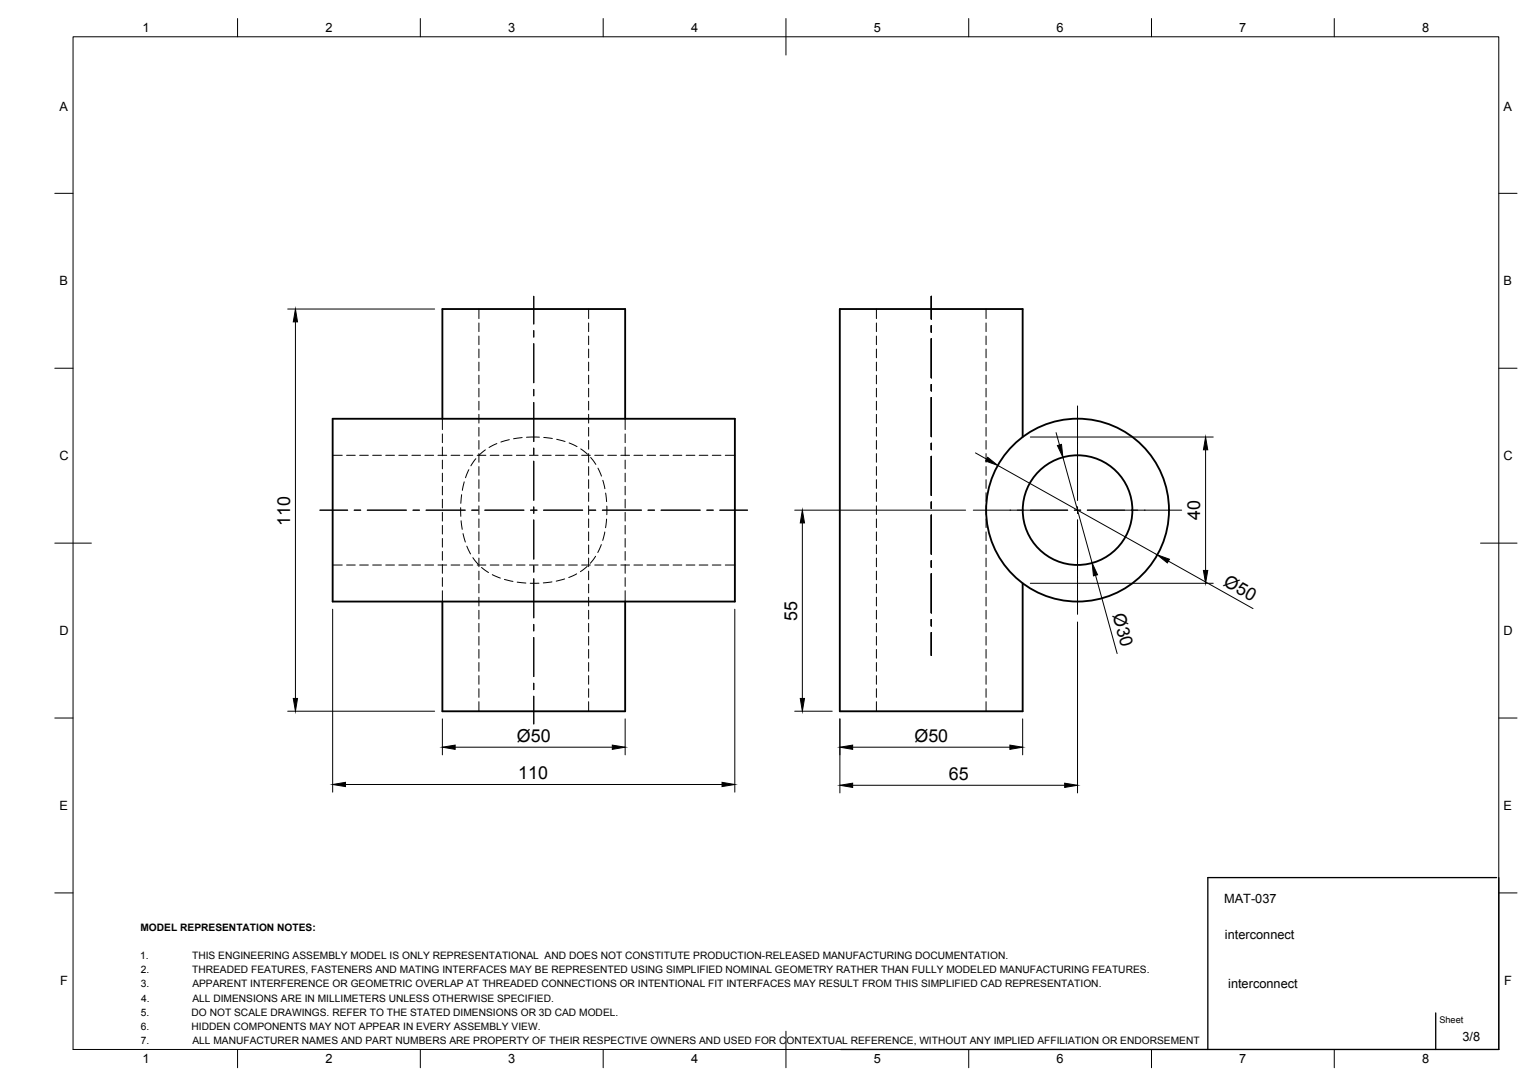
ISO-10303-21;
HEADER;
/* Generated by software containing ST-Developer
 * from STEP Tools, Inc. (www.steptools.com) 
 */

FILE_DESCRIPTION(
/* description */ ('STEP AP214'),
/* implementation_level */ '2;1');

FILE_NAME(
/* name */ 'interconnect.step',
/* time_stamp */ '2026-11-14T21:09:07-08:00',
/* author */ (''),
/* organization */ (''),
/* preprocessor_version */ 'ST-DEVELOPER v20.2',
/* originating_system */ 'Autodesk Translation Framework v15.17.0.0',
/* authorisation */ '');

FILE_SCHEMA (('AUTOMOTIVE_DESIGN { 1 0 10303 214 3 1 1 }'));
ENDSEC;

DATA;
#10=MECHANICAL_DESIGN_GEOMETRIC_PRESENTATION_REPRESENTATION('',(#78),#2059);
#64=SHAPE_REPRESENTATION_RELATIONSHIP('SRR','None',#2094,#71);
#71=ADVANCED_BREP_SHAPE_REPRESENTATION('',(#85),#2052);
#78=STYLED_ITEM('',(#2138),#85);
#85=MANIFOLD_SOLID_BREP('Body1',#975);
#92=PLANE('',#1074);
#93=PLANE('',#1075);
#94=PLANE('',#1076);
#95=PLANE('',#1077);
#125=FACE_BOUND('',#214,.T.);
#126=FACE_BOUND('',#217,.T.);
#127=FACE_BOUND('',#219,.T.);
#128=FACE_BOUND('',#221,.T.);
#129=FACE_BOUND('',#223,.T.);
#130=FACE_BOUND('',#225,.T.);
#145=B_SPLINE_CURVE_WITH_KNOTS('',3,(#1500,#1501,#1502,#1503,#1504,#1505,
#1506,#1507,#1508,#1509,#1510,#1511,#1512,#1513,#1514,#1515,#1516,#1517,
#1518,#1519,#1520,#1521,#1522,#1523,#1524,#1525,#1526,#1527,#1528,#1529,
#1530,#1531,#1532,#1533,#1534,#1535,#1536,#1537,#1538,#1539,#1540,#1541,
#1542,#1543,#1544,#1545,#1546,#1547,#1548,#1549,#1550,#1551,#1552,#1553,
#1554,#1555,#1556,#1557,#1558,#1559,#1560,#1561,#1562,#1563,#1564,#1565),
 .UNSPECIFIED.,.T.,.F.,(4,2,2,2,2,2,2,2,2,2,2,2,2,2,2,2,2,2,2,2,2,2,2,2,
2,2,2,2,2,2,2,2,4),(-13.1042885251054,-12.7312036729648,-12.3581188208242,
-11.9850339686836,-11.611949116543,-11.2858660599115,-10.95978300328,-10.3939996985545,
-9.82821639382906,-9.2624330891036,-8.69664978437814,-8.37056672774664,
-8.04448367111514,-7.67139881897453,-7.29831396683392,-6.92522911469332,
-6.55214426255271,-6.1790594104121,-5.80597455827149,-5.43288970613088,
-5.05980485399027,-4.73372179735877,-4.40763874072727,-3.84185543600181,
-3.27607213127635,-2.7102888265509,-2.14450552182544,-1.81842246519393,
-1.49233940856243,-1.11925455642182,-0.746169704281216,-0.373084852140608,
0.),.UNSPECIFIED.);
#156=FACE_OUTER_BOUND('',#212,.T.);
#157=FACE_OUTER_BOUND('',#213,.T.);
#158=FACE_OUTER_BOUND('',#215,.T.);
#159=FACE_OUTER_BOUND('',#216,.T.);
#160=FACE_OUTER_BOUND('',#218,.T.);
#161=FACE_OUTER_BOUND('',#220,.T.);
#162=FACE_OUTER_BOUND('',#222,.T.);
#163=FACE_OUTER_BOUND('',#224,.T.);
#212=EDGE_LOOP('',(#659,#660,#661,#662));
#213=EDGE_LOOP('',(#663,#664,#665,#666));
#214=EDGE_LOOP('',(#667));
#215=EDGE_LOOP('',(#668,#669,#670,#671));
#216=EDGE_LOOP('',(#672,#673,#674,#675));
#217=EDGE_LOOP('',(#676));
#218=EDGE_LOOP('',(#677));
#219=EDGE_LOOP('',(#678));
#220=EDGE_LOOP('',(#679));
#221=EDGE_LOOP('',(#680));
#222=EDGE_LOOP('',(#681));
#223=EDGE_LOOP('',(#682));
#224=EDGE_LOOP('',(#683));
#225=EDGE_LOOP('',(#684));
#288=LINE('',#1491,#353);
#289=LINE('',#1497,#354);
#290=LINE('',#1570,#355);
#291=LINE('',#1576,#356);
#353=VECTOR('',#1188,15.);
#354=VECTOR('',#1195,25.);
#355=VECTOR('',#1202,15.);
#356=VECTOR('',#1209,25.);
#418=CIRCLE('',#1063,15.);
#419=CIRCLE('',#1064,15.);
#420=CIRCLE('',#1066,25.);
#421=CIRCLE('',#1067,25.);
#422=CIRCLE('',#1069,15.);
#423=CIRCLE('',#1070,15.);
#424=CIRCLE('',#1072,25.);
#425=CIRCLE('',#1073,25.);
#461=VERTEX_POINT('',#1488);
#462=VERTEX_POINT('',#1490);
#463=VERTEX_POINT('',#1494);
#464=VERTEX_POINT('',#1496);
#465=VERTEX_POINT('',#1499);
#466=VERTEX_POINT('',#1567);
#467=VERTEX_POINT('',#1569);
#468=VERTEX_POINT('',#1573);
#469=VERTEX_POINT('',#1575);
#540=EDGE_CURVE('',#461,#461,#418,.T.);
#541=EDGE_CURVE('',#461,#462,#288,.T.);
#542=EDGE_CURVE('',#462,#462,#419,.T.);
#543=EDGE_CURVE('',#463,#463,#420,.T.);
#544=EDGE_CURVE('',#463,#464,#289,.T.);
#545=EDGE_CURVE('',#464,#464,#421,.T.);
#546=EDGE_CURVE('',#465,#465,#145,.T.);
#547=EDGE_CURVE('',#466,#466,#422,.T.);
#548=EDGE_CURVE('',#466,#467,#290,.T.);
#549=EDGE_CURVE('',#467,#467,#423,.T.);
#550=EDGE_CURVE('',#468,#468,#424,.T.);
#551=EDGE_CURVE('',#468,#469,#291,.T.);
#552=EDGE_CURVE('',#469,#469,#425,.T.);
#659=ORIENTED_EDGE('',*,*,#540,.T.);
#660=ORIENTED_EDGE('',*,*,#541,.T.);
#661=ORIENTED_EDGE('',*,*,#542,.F.);
#662=ORIENTED_EDGE('',*,*,#541,.F.);
#663=ORIENTED_EDGE('',*,*,#543,.T.);
#664=ORIENTED_EDGE('',*,*,#544,.T.);
#665=ORIENTED_EDGE('',*,*,#545,.F.);
#666=ORIENTED_EDGE('',*,*,#544,.F.);
#667=ORIENTED_EDGE('',*,*,#546,.T.);
#668=ORIENTED_EDGE('',*,*,#547,.T.);
#669=ORIENTED_EDGE('',*,*,#548,.T.);
#670=ORIENTED_EDGE('',*,*,#549,.F.);
#671=ORIENTED_EDGE('',*,*,#548,.F.);
#672=ORIENTED_EDGE('',*,*,#550,.T.);
#673=ORIENTED_EDGE('',*,*,#551,.T.);
#674=ORIENTED_EDGE('',*,*,#552,.F.);
#675=ORIENTED_EDGE('',*,*,#551,.F.);
#676=ORIENTED_EDGE('',*,*,#546,.F.);
#677=ORIENTED_EDGE('',*,*,#552,.T.);
#678=ORIENTED_EDGE('',*,*,#547,.F.);
#679=ORIENTED_EDGE('',*,*,#550,.F.);
#680=ORIENTED_EDGE('',*,*,#549,.T.);
#681=ORIENTED_EDGE('',*,*,#545,.T.);
#682=ORIENTED_EDGE('',*,*,#540,.F.);
#683=ORIENTED_EDGE('',*,*,#543,.F.);
#684=ORIENTED_EDGE('',*,*,#542,.T.);
#897=CYLINDRICAL_SURFACE('',#1062,15.);
#898=CYLINDRICAL_SURFACE('',#1065,25.);
#899=CYLINDRICAL_SURFACE('',#1068,15.);
#900=CYLINDRICAL_SURFACE('',#1071,25.);
#919=ADVANCED_FACE('',(#156),#897,.F.);
#920=ADVANCED_FACE('',(#157,#125),#898,.T.);
#921=ADVANCED_FACE('',(#158),#899,.F.);
#922=ADVANCED_FACE('',(#159,#126),#900,.T.);
#923=ADVANCED_FACE('',(#160,#127),#92,.T.);
#924=ADVANCED_FACE('',(#161,#128),#93,.F.);
#925=ADVANCED_FACE('',(#162,#129),#94,.T.);
#926=ADVANCED_FACE('',(#163,#130),#95,.F.);
#975=CLOSED_SHELL('',(#919,#920,#921,#922,#923,#924,#925,#926));
#1061=AXIS2_PLACEMENT_3D('',#1486,#1182,#1183);
#1062=AXIS2_PLACEMENT_3D('',#1487,#1184,#1185);
#1063=AXIS2_PLACEMENT_3D('',#1489,#1186,#1187);
#1064=AXIS2_PLACEMENT_3D('',#1492,#1189,#1190);
#1065=AXIS2_PLACEMENT_3D('',#1493,#1191,#1192);
#1066=AXIS2_PLACEMENT_3D('',#1495,#1193,#1194);
#1067=AXIS2_PLACEMENT_3D('',#1498,#1196,#1197);
#1068=AXIS2_PLACEMENT_3D('',#1566,#1198,#1199);
#1069=AXIS2_PLACEMENT_3D('',#1568,#1200,#1201);
#1070=AXIS2_PLACEMENT_3D('',#1571,#1203,#1204);
#1071=AXIS2_PLACEMENT_3D('',#1572,#1205,#1206);
#1072=AXIS2_PLACEMENT_3D('',#1574,#1207,#1208);
#1073=AXIS2_PLACEMENT_3D('',#1577,#1210,#1211);
#1074=AXIS2_PLACEMENT_3D('',#1578,#1212,#1213);
#1075=AXIS2_PLACEMENT_3D('',#1579,#1214,#1215);
#1076=AXIS2_PLACEMENT_3D('',#1580,#1216,#1217);
#1077=AXIS2_PLACEMENT_3D('',#1581,#1218,#1219);
#1182=DIRECTION('axis',(0.,0.,1.));
#1183=DIRECTION('refdir',(1.,0.,0.));
#1184=DIRECTION('center_axis',(0.,-1.,0.));
#1185=DIRECTION('ref_axis',(0.,0.,-1.));
#1186=DIRECTION('center_axis',(0.,1.,0.));
#1187=DIRECTION('ref_axis',(0.,0.,1.));
#1188=DIRECTION('',(0.,-1.,0.));
#1189=DIRECTION('center_axis',(0.,1.,0.));
#1190=DIRECTION('ref_axis',(0.,0.,1.));
#1191=DIRECTION('center_axis',(0.,-1.,0.));
#1192=DIRECTION('ref_axis',(0.,0.,-1.));
#1193=DIRECTION('center_axis',(0.,1.,0.));
#1194=DIRECTION('ref_axis',(0.,0.,1.));
#1195=DIRECTION('',(0.,1.,0.));
#1196=DIRECTION('center_axis',(0.,1.,0.));
#1197=DIRECTION('ref_axis',(0.,0.,1.));
#1198=DIRECTION('center_axis',(0.,0.,-1.));
#1199=DIRECTION('ref_axis',(-1.,0.,0.));
#1200=DIRECTION('center_axis',(0.,0.,1.));
#1201=DIRECTION('ref_axis',(1.,0.,0.));
#1202=DIRECTION('',(0.,0.,-1.));
#1203=DIRECTION('center_axis',(0.,0.,1.));
#1204=DIRECTION('ref_axis',(1.,0.,0.));
#1205=DIRECTION('center_axis',(0.,0.,-1.));
#1206=DIRECTION('ref_axis',(-1.,0.,0.));
#1207=DIRECTION('center_axis',(0.,0.,1.));
#1208=DIRECTION('ref_axis',(1.,0.,0.));
#1209=DIRECTION('',(0.,0.,1.));
#1210=DIRECTION('center_axis',(0.,0.,1.));
#1211=DIRECTION('ref_axis',(1.,0.,0.));
#1212=DIRECTION('center_axis',(0.,0.,1.));
#1213=DIRECTION('ref_axis',(1.,0.,0.));
#1214=DIRECTION('center_axis',(0.,0.,1.));
#1215=DIRECTION('ref_axis',(1.,0.,0.));
#1216=DIRECTION('center_axis',(0.,1.,0.));
#1217=DIRECTION('ref_axis',(0.,0.,1.));
#1218=DIRECTION('center_axis',(0.,1.,0.));
#1219=DIRECTION('ref_axis',(0.,0.,1.));
#1486=CARTESIAN_POINT('',(0.,0.,0.));
#1487=CARTESIAN_POINT('Origin',(-40.,55.,55.));
#1488=CARTESIAN_POINT('',(-40.,55.,70.));
#1489=CARTESIAN_POINT('Origin',(-40.,55.,55.));
#1490=CARTESIAN_POINT('',(-40.,-55.,70.));
#1491=CARTESIAN_POINT('',(-40.,55.,70.));
#1492=CARTESIAN_POINT('Origin',(-40.,-55.,55.));
#1493=CARTESIAN_POINT('Origin',(-40.,55.,55.));
#1494=CARTESIAN_POINT('',(-40.,-55.,80.));
#1495=CARTESIAN_POINT('Origin',(-40.,-55.,55.));
#1496=CARTESIAN_POINT('',(-40.,55.,80.));
#1497=CARTESIAN_POINT('',(-40.,55.,80.));
#1498=CARTESIAN_POINT('Origin',(-40.,55.,55.));
#1499=CARTESIAN_POINT('',(-24.9999999999999,0.,75.));
#1500=CARTESIAN_POINT('Ctrl Pts',(-25.,2.77555756156289E-16,35.));
#1501=CARTESIAN_POINT('Ctrl Pts',(-25.,-1.24361617380203,35.));
#1502=CARTESIAN_POINT('Ctrl Pts',(-24.9052472768386,-2.5300488634612,35.069860816135));
#1503=CARTESIAN_POINT('Ctrl Pts',(-24.5112512498491,-5.08635930324528,35.3744893013021));
#1504=CARTESIAN_POINT('Ctrl Pts',(-24.2120237975874,-6.35622364547916,35.6093899705556));
#1505=CARTESIAN_POINT('Ctrl Pts',(-23.4403103697305,-8.78494699666433,36.2641295306962));
#1506=CARTESIAN_POINT('Ctrl Pts',(-22.9672284001806,-9.94593352803297,36.6853433784887));
#1507=CARTESIAN_POINT('Ctrl Pts',(-21.9190504199837,-12.0818210937726,37.7193397258191));
#1508=CARTESIAN_POINT('Ctrl Pts',(-21.3446200198761,-13.0565914520077,38.3330665709257));
#1509=CARTESIAN_POINT('Ctrl Pts',(-20.2669777826776,-14.6650944479835,39.6303382528525));
#1510=CARTESIAN_POINT('Ctrl Pts',(-19.7036276546287,-15.410730934833,40.3700017631622));
#1511=CARTESIAN_POINT('Ctrl Pts',(-18.6105706812708,-16.7143714911116,42.0203271120065));
#1512=CARTESIAN_POINT('Ctrl Pts',(-18.0833825531526,-17.2737939159714,42.9315354562001));
#1513=CARTESIAN_POINT('Ctrl Pts',(-16.8688323188826,-18.4830916199472,45.3606359247402));
#1514=CARTESIAN_POINT('Ctrl Pts',(-16.1653056845286,-19.079941900497,47.1971676511035));
#1515=CARTESIAN_POINT('Ctrl Pts',(-15.2297367266376,-19.8347251545665,51.0743159129527));
#1516=CARTESIAN_POINT('Ctrl Pts',(-15.,-20.,53.1140556509152));
#1517=CARTESIAN_POINT('Ctrl Pts',(-15.,-20.,56.8859443490849));
#1518=CARTESIAN_POINT('Ctrl Pts',(-15.2297367266376,-19.8347251545665,58.9256840870473));
#1519=CARTESIAN_POINT('Ctrl Pts',(-16.1653056845286,-19.079941900497,62.8028323488965));
#1520=CARTESIAN_POINT('Ctrl Pts',(-16.8688323188826,-18.4830916199472,64.6393640752598));
#1521=CARTESIAN_POINT('Ctrl Pts',(-18.0833825531526,-17.2737939159714,67.0684645437999));
#1522=CARTESIAN_POINT('Ctrl Pts',(-18.6105706812708,-16.7143714911116,67.9796728879935));
#1523=CARTESIAN_POINT('Ctrl Pts',(-19.7036276546287,-15.410730934833,69.6299982368378));
#1524=CARTESIAN_POINT('Ctrl Pts',(-20.2669777826776,-14.6650944479835,70.3696617471475));
#1525=CARTESIAN_POINT('Ctrl Pts',(-21.3446200198761,-13.0565914520077,71.6669334290743));
#1526=CARTESIAN_POINT('Ctrl Pts',(-21.9190504199837,-12.0818210937726,72.2806602741809));
#1527=CARTESIAN_POINT('Ctrl Pts',(-22.9672284001806,-9.94593352803297,73.3146566215113));
#1528=CARTESIAN_POINT('Ctrl Pts',(-23.4403103697305,-8.78494699666433,73.7358704693038));
#1529=CARTESIAN_POINT('Ctrl Pts',(-24.2120237975874,-6.35622364547916,74.3906100294445));
#1530=CARTESIAN_POINT('Ctrl Pts',(-24.5112512498491,-5.08635930324528,74.6255106986979));
#1531=CARTESIAN_POINT('Ctrl Pts',(-24.9052472768386,-2.53004886346119,74.930139183865));
#1532=CARTESIAN_POINT('Ctrl Pts',(-25.,-1.24361617380203,75.));
#1533=CARTESIAN_POINT('Ctrl Pts',(-25.,1.24361617380203,75.));
#1534=CARTESIAN_POINT('Ctrl Pts',(-24.9052472768386,2.53004886346119,74.930139183865));
#1535=CARTESIAN_POINT('Ctrl Pts',(-24.5112512498491,5.08635930324528,74.6255106986979));
#1536=CARTESIAN_POINT('Ctrl Pts',(-24.2120237975874,6.35622364547916,74.3906100294445));
#1537=CARTESIAN_POINT('Ctrl Pts',(-23.4403103697305,8.78494699666433,73.7358704693038));
#1538=CARTESIAN_POINT('Ctrl Pts',(-22.9672284001806,9.94593352803297,73.3146566215113));
#1539=CARTESIAN_POINT('Ctrl Pts',(-21.9190504199837,12.0818210937726,72.2806602741809));
#1540=CARTESIAN_POINT('Ctrl Pts',(-21.3446200198761,13.0565914520077,71.6669334290743));
#1541=CARTESIAN_POINT('Ctrl Pts',(-20.2669777826776,14.6650944479835,70.3696617471475));
#1542=CARTESIAN_POINT('Ctrl Pts',(-19.7036276546287,15.410730934833,69.6299982368378));
#1543=CARTESIAN_POINT('Ctrl Pts',(-18.6105706812708,16.7143714911116,67.9796728879935));
#1544=CARTESIAN_POINT('Ctrl Pts',(-18.0833825531526,17.2737939159714,67.0684645437999));
#1545=CARTESIAN_POINT('Ctrl Pts',(-16.8688323188826,18.4830916199472,64.6393640752599));
#1546=CARTESIAN_POINT('Ctrl Pts',(-16.1653056845287,19.079941900497,62.8028323488965));
#1547=CARTESIAN_POINT('Ctrl Pts',(-15.2297367266376,19.8347251545665,58.9256840870473));
#1548=CARTESIAN_POINT('Ctrl Pts',(-15.,20.,56.8859443490849));
#1549=CARTESIAN_POINT('Ctrl Pts',(-15.,20.,53.1140556509151));
#1550=CARTESIAN_POINT('Ctrl Pts',(-15.2297367266376,19.8347251545665,51.0743159129527));
#1551=CARTESIAN_POINT('Ctrl Pts',(-16.1653056845287,19.079941900497,47.1971676511035));
#1552=CARTESIAN_POINT('Ctrl Pts',(-16.8688323188826,18.4830916199472,45.3606359247402));
#1553=CARTESIAN_POINT('Ctrl Pts',(-18.0833825531526,17.2737939159714,42.9315354562001));
#1554=CARTESIAN_POINT('Ctrl Pts',(-18.6105706812708,16.7143714911116,42.0203271120065));
#1555=CARTESIAN_POINT('Ctrl Pts',(-19.7036276546287,15.410730934833,40.3700017631622));
#1556=CARTESIAN_POINT('Ctrl Pts',(-20.2669777826776,14.6650944479835,39.6303382528525));
#1557=CARTESIAN_POINT('Ctrl Pts',(-21.3446200198761,13.0565914520077,38.3330665709257));
#1558=CARTESIAN_POINT('Ctrl Pts',(-21.9190504199837,12.0818210937726,37.7193397258191));
#1559=CARTESIAN_POINT('Ctrl Pts',(-22.9672284001806,9.94593352803297,36.6853433784887));
#1560=CARTESIAN_POINT('Ctrl Pts',(-23.4403103697305,8.78494699666433,36.2641295306962));
#1561=CARTESIAN_POINT('Ctrl Pts',(-24.2120237975874,6.35622364547916,35.6093899705556));
#1562=CARTESIAN_POINT('Ctrl Pts',(-24.5112512498491,5.08635930324528,35.3744893013021));
#1563=CARTESIAN_POINT('Ctrl Pts',(-24.9052472768386,2.53004886346119,35.069860816135));
#1564=CARTESIAN_POINT('Ctrl Pts',(-25.,1.24361617380203,35.));
#1565=CARTESIAN_POINT('Ctrl Pts',(-25.,-2.77555756156289E-16,35.));
#1566=CARTESIAN_POINT('Origin',(0.,0.,110.));
#1567=CARTESIAN_POINT('',(15.,-1.83697019872103E-15,110.));
#1568=CARTESIAN_POINT('Origin',(0.,0.,110.));
#1569=CARTESIAN_POINT('',(15.,-1.83697019872103E-15,0.));
#1570=CARTESIAN_POINT('',(15.,-1.83697019872103E-15,110.));
#1571=CARTESIAN_POINT('Origin',(0.,0.,0.));
#1572=CARTESIAN_POINT('Origin',(0.,0.,110.));
#1573=CARTESIAN_POINT('',(25.,-3.06161699786838E-15,0.));
#1574=CARTESIAN_POINT('Origin',(0.,0.,0.));
#1575=CARTESIAN_POINT('',(25.,-3.06161699786838E-15,110.));
#1576=CARTESIAN_POINT('',(25.,-3.06161699786838E-15,110.));
#1577=CARTESIAN_POINT('Origin',(0.,0.,110.));
#1578=CARTESIAN_POINT('Origin',(0.,0.,110.));
#1579=CARTESIAN_POINT('Origin',(0.,0.,0.));
#1580=CARTESIAN_POINT('Origin',(-40.,55.,55.));
#1581=CARTESIAN_POINT('Origin',(-40.,-55.,55.));
#2043=UNCERTAINTY_MEASURE_WITH_UNIT(LENGTH_MEASURE(0.01),#2060,
'DISTANCE_ACCURACY_VALUE',
'Maximum model space distance between geometric entities at asserted c
onnectivities');
#2050=UNCERTAINTY_MEASURE_WITH_UNIT(LENGTH_MEASURE(0.01),#2060,
'DISTANCE_ACCURACY_VALUE',
'Maximum model space distance between geometric entities at asserted c
onnectivities');
#2052=(
GEOMETRIC_REPRESENTATION_CONTEXT(3)
GLOBAL_UNCERTAINTY_ASSIGNED_CONTEXT((#2043))
GLOBAL_UNIT_ASSIGNED_CONTEXT((#2060,#2062,#2063))
REPRESENTATION_CONTEXT('','3D')
);
#2059=(
GEOMETRIC_REPRESENTATION_CONTEXT(3)
GLOBAL_UNCERTAINTY_ASSIGNED_CONTEXT((#2050))
GLOBAL_UNIT_ASSIGNED_CONTEXT((#2060,#2062,#2063))
REPRESENTATION_CONTEXT('','3D')
);
#2060=(
LENGTH_UNIT()
NAMED_UNIT(*)
SI_UNIT(.MILLI.,.METRE.)
);
#2062=(
NAMED_UNIT(*)
PLANE_ANGLE_UNIT()
SI_UNIT($,.RADIAN.)
);
#2063=(
NAMED_UNIT(*)
SI_UNIT($,.STERADIAN.)
SOLID_ANGLE_UNIT()
);
#2065=SHAPE_DEFINITION_REPRESENTATION(#2073,#2094);
#2073=PRODUCT_DEFINITION_SHAPE('',$,#2103);
#2094=SHAPE_REPRESENTATION('',(#1061),#2052);
#2101=PRODUCT_DEFINITION_CONTEXT('part definition',#2127,'design');
#2103=PRODUCT_DEFINITION('interconnect','interconnect',#2111,#2101);
#2111=PRODUCT_DEFINITION_FORMATION('',$,#2130);
#2127=APPLICATION_CONTEXT(
'Core Data for Automotive Mechanical Design Process');
#2128=PRODUCT_CONTEXT('part definition',#2127,'mechanical');
#2130=PRODUCT('interconnect','interconnect',$,(#2128));
#2138=PRESENTATION_STYLE_ASSIGNMENT((#2144));
#2144=SURFACE_STYLE_USAGE(.BOTH.,#2150);
#2150=SURFACE_SIDE_STYLE('',(#2156));
#2156=SURFACE_STYLE_FILL_AREA(#2162);
#2162=FILL_AREA_STYLE('Opaque(227,224,212)',(#2168));
#2168=FILL_AREA_STYLE_COLOUR('Opaque(227,224,212)',#2174);
#2174=COLOUR_RGB('Opaque(227,224,212)',0.890196078431372,0.87843137254902,
0.831372549019608);
ENDSEC;
END-ISO-10303-21;
